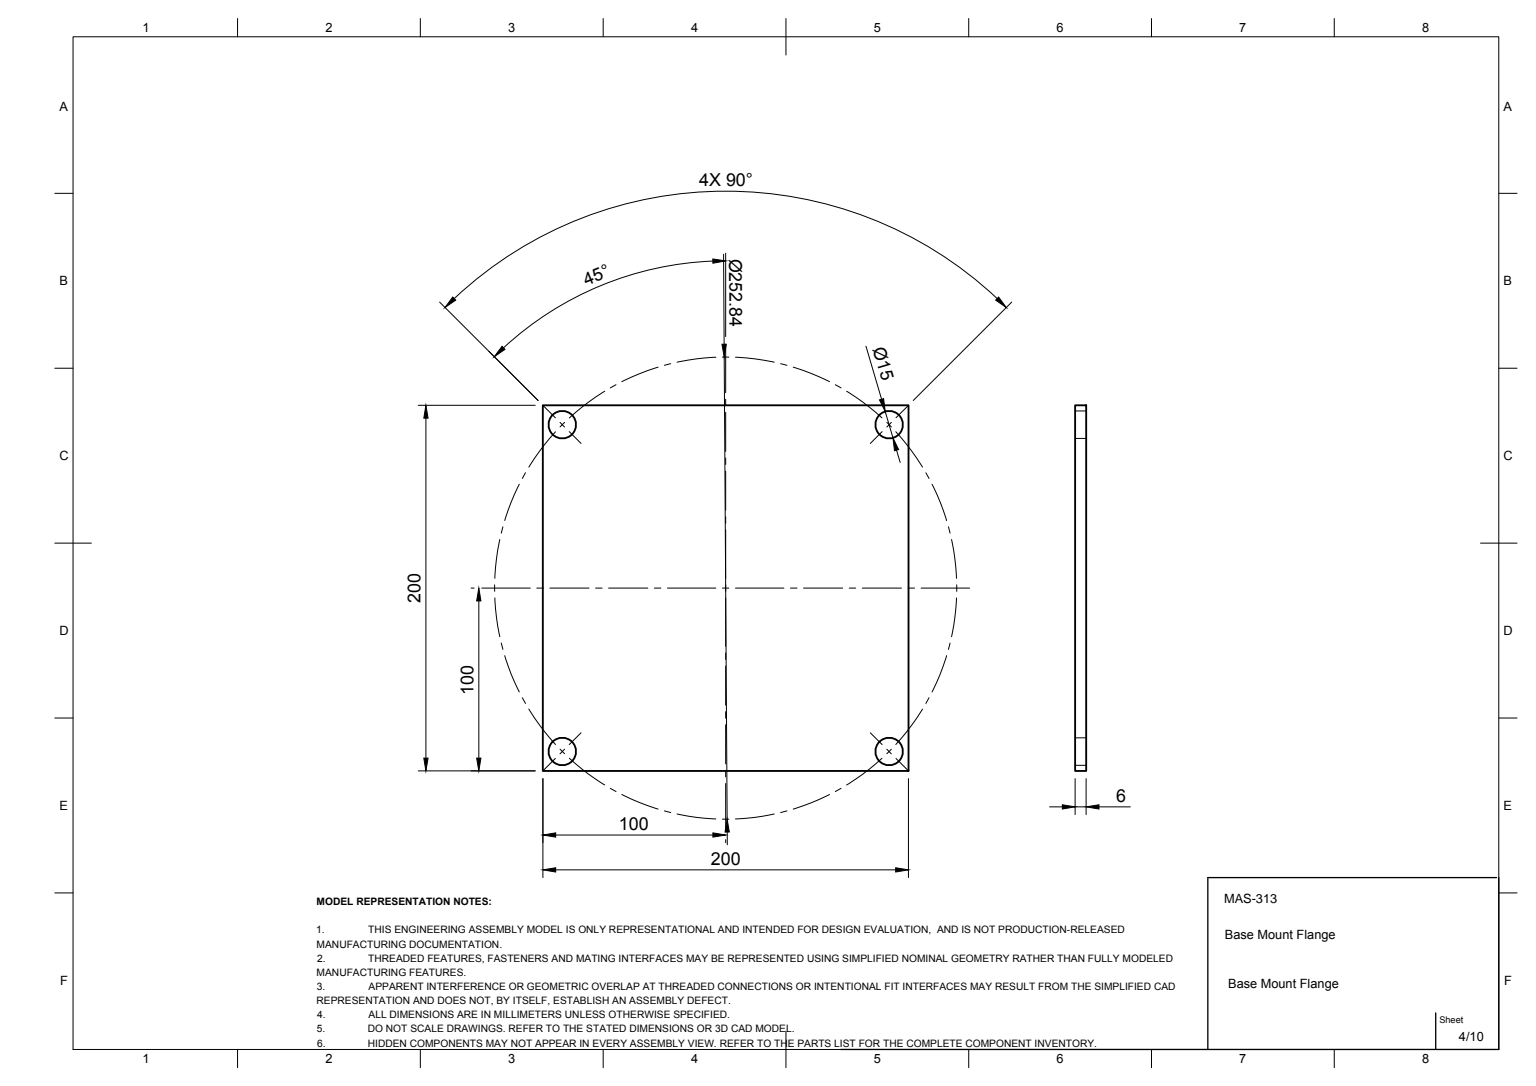
ISO-10303-21;
HEADER;
FILE_DESCRIPTION (('STEP AP214'),
    '1' );
FILE_NAME ('Base Mount Flange.step',
    '2026-10-06T09:36:00',
    ( '' ),
    ( '' ),
    'SwSTEP 2.0',
    'SolidWorks 2025',
    '' );
FILE_SCHEMA (( 'AUTOMOTIVE_DESIGN' ));
ENDSEC;

DATA;
#29=DIRECTION ( 'NONE',  ( 0.000000000000000000, 0.000000000000000000, 1.000000000000000000 ) ) ;
#31=CARTESIAN_POINT ( 'NONE',  ( 9.184850993605149917E-16, 0.000000000000000000, -133.9213562373095101 ) ) ;
#52=( NAMED_UNIT ( * ) PLANE_ANGLE_UNIT ( ) SI_UNIT ( $, .RADIAN. ) );
#69=VERTEX_POINT ( 'NONE', #7089 ) ;
#81=LINE ( 'NONE', #4059, #683 ) ;
#89=AXIS2_PLACEMENT_3D ( 'NONE', #10782, #5094, #8125 ) ;
#118=PRODUCT ( 'Base Mount Flange', 'Base Mount Flange', '', ( #4909 ) ) ;
#163=ORIENTED_EDGE ( 'NONE', *, *, #8870, .T. ) ;
#166=AXIS2_PLACEMENT_3D ( 'NONE', #11994, #9209, #3384 ) ;
#206=VERTEX_POINT ( 'NONE', #8210 ) ;
#238=EDGE_CURVE ( 'NONE', #2268, #7247, #10053, .T. ) ;
#269=DIRECTION ( 'NONE',  ( 0.000000000000000000, 0.000000000000000000, -1.000000000000000000 ) ) ;
#306=EDGE_LOOP ( 'NONE', ( #4987, #12037, #7872, #11168 ) ) ;
#325=ORIENTED_EDGE ( 'NONE', *, *, #5571, .T. ) ;
#336=LINE ( 'NONE', #1445, #8050 ) ;
#340=EDGE_CURVE ( 'NONE', #2669, #5042, #5605, .T. ) ;
#346=EDGE_LOOP ( 'NONE', ( #11443, #5040 ) ) ;
#365=ORIENTED_EDGE ( 'NONE', *, *, #10686, .T. ) ;
#368=VERTEX_POINT ( 'NONE', #31 ) ;
#387=ORIENTED_EDGE ( 'NONE', *, *, #9652, .F. ) ;
#405=CARTESIAN_POINT ( 'NONE',  ( 126.4213562373094959, -6.000000000000000000, -6.938893903907228378E-15 ) ) ;
#427=VECTOR ( 'NONE', #2802, 999.9999999999998863 ) ;
#471=ORIENTED_EDGE ( 'NONE', *, *, #4119, .T. ) ;
#534=DIRECTION ( 'NONE',  ( 0.000000000000000000, 1.000000000000000000, 0.000000000000000000 ) ) ;
#545=ORIENTED_EDGE ( 'NONE', *, *, #11311, .F. ) ;
#595=PLANE ( 'NONE',  #12120 ) ;
#617=DIRECTION ( 'NONE',  ( 0.000000000000000000, 1.000000000000000000, 0.000000000000000000 ) ) ;
#644=DIRECTION ( 'NONE',  ( 0.000000000000000000, 1.000000000000000000, 0.000000000000000000 ) ) ;
#667=CARTESIAN_POINT ( 'NONE',  ( -126.4213562373094959, -6.000000000000000000, -7.499999999999990230 ) ) ;
#683=VECTOR ( 'NONE', #11412, 1000.000000000000000 ) ;
#699=FACE_OUTER_BOUND ( 'NONE', #2730, .T. ) ;
#703=DIRECTION ( 'NONE',  ( -0.7071067811865479058, 0.000000000000000000, -0.7071067811865472397 ) ) ;
#715=CARTESIAN_POINT ( 'NONE',  ( 4.808665244885994618E-14, -6.000000000000000000, 141.4213562373094817 ) ) ;
#729=VECTOR ( 'NONE', #2030, 1000.000000000000000 ) ;
#742=CARTESIAN_POINT ( 'NONE',  ( 126.4213562373094959, -6.000000000000000000, -6.938893903907228378E-15 ) ) ;
#760=AXIS2_PLACEMENT_3D ( 'NONE', #9887, #5181, #11805 ) ;
#769=PLANE ( 'NONE',  #3066 ) ;
#771=PLANE ( 'NONE',  #1682 ) ;
#809=EDGE_LOOP ( 'NONE', ( #4329, #2289, #4115, #6023 ) ) ;
#811=CARTESIAN_POINT ( 'NONE',  ( 1.387778780781445676E-14, -6.000000000000000000, 126.4213562373094959 ) ) ;
#815=SURFACE_STYLE_FILL_AREA ( #9277 ) ;
#883=DIRECTION ( 'NONE',  ( 0.000000000000000000, 0.000000000000000000, -1.000000000000000000 ) ) ;
#885=CIRCLE ( 'NONE', #12132, 7.500000000000007105 ) ;
#951=ORIENTED_EDGE ( 'NONE', *, *, #3247, .T. ) ;
#967=VECTOR ( 'NONE', #6992, 999.9999999999998863 ) ;
#1130=VECTOR ( 'NONE', #12111, 1000.000000000000000 ) ;
#1133=EDGE_LOOP ( 'NONE', ( #5075, #8034, #10647, #2735 ) ) ;
#1141=ORIENTED_EDGE ( 'NONE', *, *, #8393, .T. ) ;
#1168=ADVANCED_FACE ( 'NONE', ( #10376 ), #7419, .F. ) ;
#1189=CIRCLE ( 'NONE', #4922, 7.500000000000007105 ) ;
#1219=VERTEX_POINT ( 'NONE', #9205 ) ;
#1274=AXIS2_PLACEMENT_3D ( 'NONE', #10202, #9278, #11130 ) ;
#1284=CIRCLE ( 'NONE', #89, 7.500000000000007105 ) ;
#1296=CYLINDRICAL_SURFACE ( 'NONE', #1870, 7.500000000000007105 ) ;
#1328=CARTESIAN_POINT ( 'NONE',  ( 4.808665244885994618E-14, 0.000000000000000000, 141.4213562373094817 ) ) ;
#1372=CIRCLE ( 'NONE', #166, 7.500000000000012434 ) ;
#1377=ADVANCED_FACE ( 'NONE', ( #9751 ), #1296, .F. ) ;
#1410=DIRECTION ( 'NONE',  ( 0.000000000000000000, 0.000000000000000000, 1.000000000000000000 ) ) ;
#1414=VERTEX_POINT ( 'NONE', #5983 ) ;
#1415=DIRECTION ( 'NONE',  ( 0.000000000000000000, 1.000000000000000000, 0.000000000000000000 ) ) ;
#1436=ORIENTED_EDGE ( 'NONE', *, *, #10649, .T. ) ;
#1445=CARTESIAN_POINT ( 'NONE',  ( 141.4213562373095101, -6.000000000000000000, -1.508194112741312283E-14 ) ) ;
#1629=FACE_OUTER_BOUND ( 'NONE', #9194, .T. ) ;
#1682=AXIS2_PLACEMENT_3D ( 'NONE', #5167, #3665, #703 ) ;
#1685=ADVANCED_FACE ( 'NONE', ( #9060 ), #595, .T. ) ;
#1690=VERTEX_POINT ( 'NONE', #10112 ) ;
#1794=EDGE_CURVE ( 'NONE', #6737, #10573, #4624, .T. ) ;
#1796=DIRECTION ( 'NONE',  ( 0.000000000000000000, 0.000000000000000000, 1.000000000000000000 ) ) ;
#1804=FACE_BOUND ( 'NONE', #4441, .T. ) ;
#1819=DIRECTION ( 'NONE',  ( 0.000000000000000000, 0.000000000000000000, 1.000000000000000000 ) ) ;
#1822=ORIENTED_EDGE ( 'NONE', *, *, #2939, .F. ) ;
#1828=DIRECTION ( 'NONE',  ( 0.000000000000000000, 0.000000000000000000, 1.000000000000000000 ) ) ;
#1835=VERTEX_POINT ( 'NONE', #2767 ) ;
#1851=CARTESIAN_POINT ( 'NONE',  ( -141.4213562373095101, 0.000000000000000000, 3.644282033693712520E-14 ) ) ;
#1870=AXIS2_PLACEMENT_3D ( 'NONE', #5794, #2163, #7715 ) ;
#1927=CIRCLE ( 'NONE', #5071, 7.500000000000012434 ) ;
#1946=ADVANCED_FACE ( 'NONE', ( #11248 ), #2636, .T. ) ;
#1961=CARTESIAN_POINT ( 'NONE',  ( 0.000000000000000000, -6.000000000000000000, -126.4213562373094959 ) ) ;
#2030=DIRECTION ( 'NONE',  ( 0.000000000000000000, 1.000000000000000000, 0.000000000000000000 ) ) ;
#2032=SHAPE_REPRESENTATION ( 'Base Mount Flange', ( #11957 ), #5231 ) ;
#2073=VERTEX_POINT ( 'NONE', #11418 ) ;
#2095=ORIENTED_EDGE ( 'NONE', *, *, #5571, .F. ) ;
#2107=CARTESIAN_POINT ( 'NONE',  ( 9.184850993605149917E-16, -6.000000000000000000, -133.9213562373095101 ) ) ;
#2136=CARTESIAN_POINT ( 'NONE',  ( 141.4213562373095101, 0.000000000000000000, -1.508194112741312283E-14 ) ) ;
#2163=DIRECTION ( 'NONE',  ( 0.000000000000000000, 1.000000000000000000, 0.000000000000000000 ) ) ;
#2173=VECTOR ( 'NONE', #8279, 1000.000000000000000 ) ;
#2217=DIRECTION ( 'NONE',  ( 0.000000000000000000, 1.000000000000000000, 0.000000000000000000 ) ) ;
#2252=ORIENTED_EDGE ( 'NONE', *, *, #3563, .F. ) ;
#2268=VERTEX_POINT ( 'NONE', #7013 ) ;
#2289=ORIENTED_EDGE ( 'NONE', *, *, #3136, .T. ) ;
#2296=LINE ( 'NONE', #4155, #967 ) ;
#2311=LINE ( 'NONE', #6080, #8141 ) ;
#2328=ORIENTED_EDGE ( 'NONE', *, *, #238, .T. ) ;
#2431=DIRECTION ( 'NONE',  ( -0.7071067811865479058, 0.000000000000000000, -0.7071067811865472397 ) ) ;
#2462=DIRECTION ( 'NONE',  ( 0.000000000000000000, 1.000000000000000000, 0.000000000000000000 ) ) ;
#2505=CARTESIAN_POINT ( 'NONE',  ( -126.4213562373094959, -6.000000000000000000, 2.255140518769849223E-14 ) ) ;
#2566=CYLINDRICAL_SURFACE ( 'NONE', #4120, 7.500000000000012434 ) ;
#2587=LINE ( 'NONE', #12124, #11929 ) ;
#2599=LINE ( 'NONE', #5733, #729 ) ;
#2629=CARTESIAN_POINT ( 'NONE',  ( 126.4213562373094959, -6.000000000000000000, 7.500000000000006217 ) ) ;
#2636=PLANE ( 'NONE',  #6970 ) ;
#2663=ORIENTED_EDGE ( 'NONE', *, *, #9249, .F. ) ;
#2669=VERTEX_POINT ( 'NONE', #9123 ) ;
#2676=DIRECTION ( 'NONE',  ( -0.7071067811865473507, 0.000000000000000000, 0.7071067811865477948 ) ) ;
#2711=CARTESIAN_POINT ( 'NONE',  ( 126.4213562373094959, -6.000000000000000000, 7.500000000000006217 ) ) ;
#2714=VECTOR ( 'NONE', #1415, 1000.000000000000000 ) ;
#2723=CARTESIAN_POINT ( 'NONE',  ( 0.000000000000000000, 0.000000000000000000, -126.4213562373094959 ) ) ;
#2730=EDGE_LOOP ( 'NONE', ( #5594, #2095, #163, #11247 ) ) ;
#2735=ORIENTED_EDGE ( 'NONE', *, *, #11986, .F. ) ;
#2754=DIRECTION ( 'NONE',  ( 0.000000000000000000, 1.000000000000000000, 0.000000000000000000 ) ) ;
#2762=EDGE_LOOP ( 'NONE', ( #10234, #2252 ) ) ;
#2767=CARTESIAN_POINT ( 'NONE',  ( -126.4213562373094959, -6.000000000000000000, -7.499999999999990230 ) ) ;
#2802=DIRECTION ( 'NONE',  ( -0.7071067811865473507, -0.000000000000000000, 0.7071067811865477948 ) ) ;
#2807=VECTOR ( 'NONE', #2462, 1000.000000000000000 ) ;
#2846=DIRECTION ( 'NONE',  ( 0.000000000000000000, 0.000000000000000000, 1.000000000000000000 ) ) ;
#2939=EDGE_CURVE ( 'NONE', #206, #8172, #3231, .T. ) ;
#3065=FACE_BOUND ( 'NONE', #5038, .T. ) ;
#3066=AXIS2_PLACEMENT_3D ( 'NONE', #11833, #5521, #2676 ) ;
#3084=CARTESIAN_POINT ( 'NONE',  ( -6.360897667028196044E-14, 0.000000000000000000, -141.4213562373094817 ) ) ;
#3136=EDGE_CURVE ( 'NONE', #69, #7247, #2587, .T. ) ;
#3155=EDGE_CURVE ( 'NONE', #7478, #12001, #7190, .T. ) ;
#3231=CIRCLE ( 'NONE', #6397, 7.500000000000007105 ) ;
#3247=EDGE_CURVE ( 'NONE', #1219, #5163, #7881, .T. ) ;
#3250=VECTOR ( 'NONE', #10946, 1000.000000000000000 ) ;
#3347=ORIENTED_EDGE ( 'NONE', *, *, #6546, .T. ) ;
#3384=DIRECTION ( 'NONE',  ( 0.000000000000000000, 0.000000000000000000, 1.000000000000000000 ) ) ;
#3407=CARTESIAN_POINT ( 'NONE',  ( 1.387778780781445676E-14, -6.000000000000000000, 133.9213562373095101 ) ) ;
#3415=ADVANCED_FACE ( 'NONE', ( #4015 ), #11558, .F. ) ;
#3434=VERTEX_POINT ( 'NONE', #3084 ) ;
#3475=DIRECTION ( 'NONE',  ( 0.000000000000000000, 1.000000000000000000, 0.000000000000000000 ) ) ;
#3495=ORIENTED_EDGE ( 'NONE', *, *, #4816, .F. ) ;
#3527=FACE_OUTER_BOUND ( 'NONE', #5714, .T. ) ;
#3534=DIRECTION ( 'NONE',  ( 0.000000000000000000, 0.000000000000000000, 1.000000000000000000 ) ) ;
#3550=ADVANCED_FACE ( 'NONE', ( #10986 ), #9752, .F. ) ;
#3563=EDGE_CURVE ( 'NONE', #1690, #5876, #6103, .T. ) ;
#3572=FACE_BOUND ( 'NONE', #2762, .T. ) ;
#3638=PRESENTATION_STYLE_ASSIGNMENT (( #8363 ) ) ;
#3665=DIRECTION ( 'NONE',  ( 0.7071067811865472397, 0.000000000000000000, -0.7071067811865479058 ) ) ;
#3670=PRODUCT_DEFINITION_FORMATION_WITH_SPECIFIED_SOURCE ( 'ANY', '', #118, .NOT_KNOWN. ) ;
#3691=EDGE_LOOP ( 'NONE', ( #9564, #6137, #10492, #8006 ) ) ;
#3709=CARTESIAN_POINT ( 'NONE',  ( -126.4213562373094959, -6.000000000000000000, 7.500000000000035527 ) ) ;
#3763=ORIENTED_EDGE ( 'NONE', *, *, #3155, .T. ) ;
#3769=( NAMED_UNIT ( * ) SI_UNIT ( $, .STERADIAN. ) SOLID_ANGLE_UNIT ( ) );
#3801=ORIENTED_EDGE ( 'NONE', *, *, #4816, .T. ) ;
#3803=EDGE_CURVE ( 'NONE', #5876, #1690, #5511, .T. ) ;
#3822=EDGE_CURVE ( 'NONE', #12001, #7478, #1372, .T. ) ;
#3860=MANIFOLD_SOLID_BREP ( 'Boss-Extrude1', #8083 ) ;
#3934=CARTESIAN_POINT ( 'NONE',  ( 0.000000000000000000, -6.000000000000000000, 0.000000000000000000 ) ) ;
#3960=ORIENTED_EDGE ( 'NONE', *, *, #10605, .F. ) ;
#3961=ORIENTED_EDGE ( 'NONE', *, *, #1794, .F. ) ;
#4015=FACE_OUTER_BOUND ( 'NONE', #7902, .T. ) ;
#4034=CIRCLE ( 'NONE', #1274, 7.500000000000012434 ) ;
#4059=CARTESIAN_POINT ( 'NONE',  ( 9.184850993605153861E-16, -6.000000000000000000, -133.9213562373095101 ) ) ;
#4071=ORIENTED_EDGE ( 'NONE', *, *, #4965, .T. ) ;
#4115=ORIENTED_EDGE ( 'NONE', *, *, #5783, .T. ) ;
#4119=EDGE_CURVE ( 'NONE', #10573, #6737, #1189, .T. ) ;
#4120=AXIS2_PLACEMENT_3D ( 'NONE', #2505, #7209, #7399 ) ;
#4155=CARTESIAN_POINT ( 'NONE',  ( -141.4213562373095101, -6.000000000000000000, 3.644282033693712520E-14 ) ) ;
#4161=DIRECTION ( 'NONE',  ( 0.000000000000000000, 1.000000000000000000, 0.000000000000000000 ) ) ;
#4163=ORIENTED_EDGE ( 'NONE', *, *, #11692, .T. ) ;
#4329=ORIENTED_EDGE ( 'NONE', *, *, #7278, .T. ) ;
#4361=ADVANCED_FACE ( 'NONE', ( #7270 ), #2566, .F. ) ;
#4394=FACE_BOUND ( 'NONE', #11723, .T. ) ;
#4441=EDGE_LOOP ( 'NONE', ( #6502, #4537 ) ) ;
#4464=CARTESIAN_POINT ( 'NONE',  ( -126.4213562373094959, 0.000000000000000000, -7.499999999999990230 ) ) ;
#4475=CIRCLE ( 'NONE', #11381, 7.500000000000012434 ) ;
#4493=CIRCLE ( 'NONE', #7846, 7.500000000000012434 ) ;
#4520=DIRECTION ( 'NONE',  ( 0.000000000000000000, 1.000000000000000000, 0.000000000000000000 ) ) ;
#4537=ORIENTED_EDGE ( 'NONE', *, *, #6350, .F. ) ;
#4587=SURFACE_SIDE_STYLE ('',( #815 ) ) ;
#4599=ADVANCED_FACE ( 'NONE', ( #4746 ), #4912, .F. ) ;
#4624=CIRCLE ( 'NONE', #11521, 7.500000000000007105 ) ;
#4746=FACE_OUTER_BOUND ( 'NONE', #9447, .T. ) ;
#4759=CARTESIAN_POINT ( 'NONE',  ( 0.000000000000000000, -6.000000000000000000, -126.4213562373094959 ) ) ;
#4777=DIRECTION ( 'NONE',  ( 0.000000000000000000, 0.000000000000000000, 1.000000000000000000 ) ) ;
#4816=EDGE_CURVE ( 'NONE', #5163, #7478, #5475, .T. ) ;
#4823=AXIS2_PLACEMENT_3D ( 'NONE', #9717, #5069, #5011 ) ;
#4854=PLANE ( 'NONE',  #6567 ) ;
#4906=DIRECTION ( 'NONE',  ( 0.7071067811865479058, -0.000000000000000000, 0.7071067811865472397 ) ) ;
#4909=PRODUCT_CONTEXT ( 'NONE', #9295, 'mechanical' ) ;
#4912=CYLINDRICAL_SURFACE ( 'NONE', #9238, 7.500000000000007105 ) ;
#4914=FACE_OUTER_BOUND ( 'NONE', #1133, .T. ) ;
#4922=AXIS2_PLACEMENT_3D ( 'NONE', #9968, #7060, #10831 ) ;
#4951=ORIENTED_EDGE ( 'NONE', *, *, #11986, .T. ) ;
#4965=EDGE_CURVE ( 'NONE', #1219, #12001, #6919, .T. ) ;
#4974=UNCERTAINTY_MEASURE_WITH_UNIT (LENGTH_MEASURE( 1.000000000000000082E-05 ), #8426, 'distance_accuracy_value', 'NONE');
#4977=AXIS2_PLACEMENT_3D ( 'NONE', #11946, #7318, #1819 ) ;
#4982=ORIENTED_EDGE ( 'NONE', *, *, #6350, .T. ) ;
#4987=ORIENTED_EDGE ( 'NONE', *, *, #7278, .F. ) ;
#5011=DIRECTION ( 'NONE',  ( 0.000000000000000000, 0.000000000000000000, 1.000000000000000000 ) ) ;
#5018=CARTESIAN_POINT ( 'NONE',  ( -126.4213562373094959, 0.000000000000000000, 2.255140518769849223E-14 ) ) ;
#5038=EDGE_LOOP ( 'NONE', ( #1141, #5808 ) ) ;
#5040=ORIENTED_EDGE ( 'NONE', *, *, #2939, .T. ) ;
#5042=VERTEX_POINT ( 'NONE', #8037 ) ;
#5057=DIRECTION ( 'NONE',  ( 0.000000000000000000, 1.000000000000000000, 0.000000000000000000 ) ) ;
#5069=DIRECTION ( 'NONE',  ( 0.000000000000000000, 1.000000000000000000, 0.000000000000000000 ) ) ;
#5071=AXIS2_PLACEMENT_3D ( 'NONE', #11029, #10100, #1828 ) ;
#5075=ORIENTED_EDGE ( 'NONE', *, *, #340, .F. ) ;
#5094=DIRECTION ( 'NONE',  ( 0.000000000000000000, 1.000000000000000000, 0.000000000000000000 ) ) ;
#5101=AXIS2_PLACEMENT_3D ( 'NONE', #11005, #6309, #883 ) ;
#5108=AXIS2_PLACEMENT_3D ( 'NONE', #4759, #2217, #6912 ) ;
#5161=ORIENTED_EDGE ( 'NONE', *, *, #4119, .F. ) ;
#5163=VERTEX_POINT ( 'NONE', #2711 ) ;
#5167=CARTESIAN_POINT ( 'NONE',  ( 141.4213562373095101, -6.000000000000000000, -1.508194112741312283E-14 ) ) ;
#5177=DIRECTION ( 'NONE',  ( 0.000000000000000000, 1.000000000000000000, 0.000000000000000000 ) ) ;
#5181=DIRECTION ( 'NONE',  ( 0.000000000000000000, 1.000000000000000000, 0.000000000000000000 ) ) ;
#5231=( GEOMETRIC_REPRESENTATION_CONTEXT ( 3 ) GLOBAL_UNCERTAINTY_ASSIGNED_CONTEXT ( ( #6835 ) ) GLOBAL_UNIT_ASSIGNED_CONTEXT ( ( #7077, #7202, #5973 ) ) REPRESENTATION_CONTEXT ( 'NONE', 'WORKASPACE' ) );
#5448=ORIENTED_EDGE ( 'NONE', *, *, #1794, .T. ) ;
#5475=LINE ( 'NONE', #2629, #7131 ) ;
#5494=EDGE_LOOP ( 'NONE', ( #11595, #3960, #4951, #2328 ) ) ;
#5511=CIRCLE ( 'NONE', #12235, 7.500000000000007105 ) ;
#5516=ORIENTED_EDGE ( 'NONE', *, *, #10153, .T. ) ;
#5521=DIRECTION ( 'NONE',  ( -0.7071067811865477948, 0.000000000000000000, -0.7071067811865473507 ) ) ;
#5536=LINE ( 'NONE', #11237, #11392 ) ;
#5540=DIRECTION ( 'NONE',  ( -0.7071067811865472397, 0.000000000000000000, 0.7071067811865479058 ) ) ;
#5551=EDGE_LOOP ( 'NONE', ( #11276, #10366, #9344, #2663 ) ) ;
#5571=EDGE_CURVE ( 'NONE', #5951, #3434, #8098, .T. ) ;
#5594=ORIENTED_EDGE ( 'NONE', *, *, #5948, .F. ) ;
#5605=LINE ( 'NONE', #7403, #6512 ) ;
#5609=DIRECTION ( 'NONE',  ( 0.7071067811865477948, -0.000000000000000000, 0.7071067811865473507 ) ) ;
#5695=ADVANCED_FACE ( 'NONE', ( #3065, #6768, #9678, #10542, #4914 ), #4854, .T. ) ;
#5714=EDGE_LOOP ( 'NONE', ( #8458, #4071, #9918, #3495 ) ) ;
#5733=CARTESIAN_POINT ( 'NONE',  ( 1.479627290717497352E-14, -6.000000000000000000, 118.9213562373094817 ) ) ;
#5737=EDGE_LOOP ( 'NONE', ( #471, #5448 ) ) ;
#5783=EDGE_CURVE ( 'NONE', #7247, #3434, #2311, .T. ) ;
#5794=CARTESIAN_POINT ( 'NONE',  ( 1.387778780781445676E-14, -6.000000000000000000, 126.4213562373094959 ) ) ;
#5808=ORIENTED_EDGE ( 'NONE', *, *, #6542, .T. ) ;
#5876=VERTEX_POINT ( 'NONE', #10031 ) ;
#5896=AXIS2_PLACEMENT_3D ( 'NONE', #742, #4520, #2846 ) ;
#5932=CYLINDRICAL_SURFACE ( 'NONE', #8048, 7.500000000000012434 ) ;
#5933=ADVANCED_FACE ( 'NONE', ( #3527 ), #12008, .F. ) ;
#5939=EDGE_LOOP ( 'NONE', ( #10719, #387 ) ) ;
#5948=EDGE_CURVE ( 'NONE', #3434, #8433, #8179, .T. ) ;
#5951=VERTEX_POINT ( 'NONE', #11017 ) ;
#5973=( NAMED_UNIT ( * ) SI_UNIT ( $, .STERADIAN. ) SOLID_ANGLE_UNIT ( ) );
#5983=CARTESIAN_POINT ( 'NONE',  ( 0.000000000000000000, 0.000000000000000000, -118.9213562373094817 ) ) ;
#6023=ORIENTED_EDGE ( 'NONE', *, *, #5948, .T. ) ;
#6080=CARTESIAN_POINT ( 'NONE',  ( 141.4213562373095101, 0.000000000000000000, -1.508194112741312283E-14 ) ) ;
#6103=CIRCLE ( 'NONE', #6884, 7.500000000000007105 ) ;
#6113=CARTESIAN_POINT ( 'NONE',  ( 1.387778780781445676E-14, 0.000000000000000000, 126.4213562373094959 ) ) ;
#6137=ORIENTED_EDGE ( 'NONE', *, *, #8393, .F. ) ;
#6307=CARTESIAN_POINT ( 'NONE',  ( 0.000000000000000000, -6.000000000000000000, -118.9213562373094817 ) ) ;
#6308=ORIENTED_EDGE ( 'NONE', *, *, #5783, .F. ) ;
#6309=DIRECTION ( 'NONE',  ( 0.000000000000000000, -1.000000000000000000, 0.000000000000000000 ) ) ;
#6333=CARTESIAN_POINT ( 'NONE',  ( 126.4213562373094959, 0.000000000000000000, -7.500000000000019540 ) ) ;
#6338=DIRECTION ( 'NONE',  ( 0.000000000000000000, 0.000000000000000000, 1.000000000000000000 ) ) ;
#6350=EDGE_CURVE ( 'NONE', #368, #1414, #11333, .T. ) ;
#6397=AXIS2_PLACEMENT_3D ( 'NONE', #7373, #9291, #4777 ) ;
#6502=ORIENTED_EDGE ( 'NONE', *, *, #6546, .F. ) ;
#6512=VECTOR ( 'NONE', #9382, 999.9999999999998863 ) ;
#6542=EDGE_CURVE ( 'NONE', #1835, #11782, #4034, .T. ) ;
#6546=EDGE_CURVE ( 'NONE', #1414, #368, #885, .T. ) ;
#6567=AXIS2_PLACEMENT_3D ( 'NONE', #3934, #7763, #269 ) ;
#6592=CARTESIAN_POINT ( 'NONE',  ( 0.000000000000000000, -6.000000000000000000, -126.4213562373094959 ) ) ;
#6605=AXIS2_PLACEMENT_3D ( 'NONE', #12189, #10131, #1796 ) ;
#6635=ORIENTED_EDGE ( 'NONE', *, *, #11042, .T. ) ;
#6737=VERTEX_POINT ( 'NONE', #2107 ) ;
#6768=FACE_BOUND ( 'NONE', #346, .T. ) ;
#6835=UNCERTAINTY_MEASURE_WITH_UNIT (LENGTH_MEASURE( 1.000000000000000082E-05 ), #7077, 'distance_accuracy_value', 'NONE');
#6884=AXIS2_PLACEMENT_3D ( 'NONE', #6113, #534, #1410 ) ;
#6894=( GEOMETRIC_REPRESENTATION_CONTEXT ( 3 ) GLOBAL_UNCERTAINTY_ASSIGNED_CONTEXT ( ( #4974 ) ) GLOBAL_UNIT_ASSIGNED_CONTEXT ( ( #8426, #52, #3769 ) ) REPRESENTATION_CONTEXT ( 'NONE', 'WORKASPACE' ) );
#6912=DIRECTION ( 'NONE',  ( 0.000000000000000000, 0.000000000000000000, 1.000000000000000000 ) ) ;
#6919=LINE ( 'NONE', #11685, #10691 ) ;
#6945=DIRECTION ( 'NONE',  ( -0.7071067811865479058, 0.000000000000000000, -0.7071067811865472397 ) ) ;
#6957=CARTESIAN_POINT ( 'NONE',  ( 4.808665244885994618E-14, -6.000000000000000000, 141.4213562373094817 ) ) ;
#6970=AXIS2_PLACEMENT_3D ( 'NONE', #9256, #5609, #9385 ) ;
#6992=DIRECTION ( 'NONE',  ( -0.7071067811865473507, -0.000000000000000000, 0.7071067811865477948 ) ) ;
#7013=CARTESIAN_POINT ( 'NONE',  ( 141.4213562373095101, -6.000000000000000000, -1.508194112741312283E-14 ) ) ;
#7060=DIRECTION ( 'NONE',  ( 0.000000000000000000, 1.000000000000000000, 0.000000000000000000 ) ) ;
#7077=( LENGTH_UNIT ( ) NAMED_UNIT ( * ) SI_UNIT ( .MILLI., .METRE. ) );
#7089=CARTESIAN_POINT ( 'NONE',  ( 4.808665244885994618E-14, 0.000000000000000000, 141.4213562373094817 ) ) ;
#7099=LINE ( 'NONE', #9884, #2714 ) ;
#7131=VECTOR ( 'NONE', #7150, 1000.000000000000000 ) ;
#7144=DIRECTION ( 'NONE',  ( 0.7071067811865473507, 0.000000000000000000, -0.7071067811865477948 ) ) ;
#7150=DIRECTION ( 'NONE',  ( 0.000000000000000000, 1.000000000000000000, 0.000000000000000000 ) ) ;
#7158=APPLICATION_CONTEXT ( 'automotive_design' ) ;
#7161=FACE_OUTER_BOUND ( 'NONE', #5551, .T. ) ;
#7186=EDGE_LOOP ( 'NONE', ( #1822, #5516, #12129, #9492 ) ) ;
#7190=CIRCLE ( 'NONE', #6605, 7.500000000000012434 ) ;
#7202=( NAMED_UNIT ( * ) PLANE_ANGLE_UNIT ( ) SI_UNIT ( $, .RADIAN. ) );
#7209=DIRECTION ( 'NONE',  ( 0.000000000000000000, 1.000000000000000000, 0.000000000000000000 ) ) ;
#7236=DIRECTION ( 'NONE',  ( 0.000000000000000000, 0.000000000000000000, 1.000000000000000000 ) ) ;
#7247=VERTEX_POINT ( 'NONE', #2136 ) ;
#7252=CARTESIAN_POINT ( 'NONE',  ( -141.4213562373095101, 0.000000000000000000, 3.644282033693712520E-14 ) ) ;
#7270=FACE_OUTER_BOUND ( 'NONE', #3691, .T. ) ;
#7278=EDGE_CURVE ( 'NONE', #8433, #69, #7755, .T. ) ;
#7318=DIRECTION ( 'NONE',  ( 0.000000000000000000, 1.000000000000000000, 0.000000000000000000 ) ) ;
#7373=CARTESIAN_POINT ( 'NONE',  ( 1.387778780781445676E-14, -6.000000000000000000, 126.4213562373094959 ) ) ;
#7399=DIRECTION ( 'NONE',  ( 0.000000000000000000, 0.000000000000000000, 1.000000000000000000 ) ) ;
#7403=CARTESIAN_POINT ( 'NONE',  ( 4.808665244885994618E-14, -6.000000000000000000, 141.4213562373094817 ) ) ;
#7419=CYLINDRICAL_SURFACE ( 'NONE', #7549, 7.500000000000007105 ) ;
#7478=VERTEX_POINT ( 'NONE', #10459 ) ;
#7493=STYLED_ITEM ( 'NONE', ( #3638 ), #3860 ) ;
#7549=AXIS2_PLACEMENT_3D ( 'NONE', #811, #9455, #9272 ) ;
#7643=ADVANCED_FACE ( 'NONE', ( #1629 ), #771, .T. ) ;
#7649=VECTOR ( 'NONE', #2754, 1000.000000000000000 ) ;
#7715=DIRECTION ( 'NONE',  ( 0.000000000000000000, 0.000000000000000000, 1.000000000000000000 ) ) ;
#7722=EDGE_LOOP ( 'NONE', ( #12009, #10107, #3801, #3763 ) ) ;
#7743=ORIENTED_EDGE ( 'NONE', *, *, #11042, .F. ) ;
#7744=ADVANCED_FACE ( 'NONE', ( #699 ), #769, .T. ) ;
#7755=LINE ( 'NONE', #1328, #7799 ) ;
#7763=DIRECTION ( 'NONE',  ( 0.000000000000000000, -1.000000000000000000, 0.000000000000000000 ) ) ;
#7799=VECTOR ( 'NONE', #4906, 999.9999999999998863 ) ;
#7846=AXIS2_PLACEMENT_3D ( 'NONE', #11092, #3475, #3534 ) ;
#7872=ORIENTED_EDGE ( 'NONE', *, *, #340, .T. ) ;
#7876=DIRECTION ( 'NONE',  ( 0.000000000000000000, 0.000000000000000000, 1.000000000000000000 ) ) ;
#7881=CIRCLE ( 'NONE', #5896, 7.500000000000012434 ) ;
#7902=EDGE_LOOP ( 'NONE', ( #3961, #6635, #4982, #11844 ) ) ;
#7955=DIRECTION ( 'NONE',  ( 1.000000000000000000, 0.000000000000000000, 0.000000000000000000 ) ) ;
#8006=ORIENTED_EDGE ( 'NONE', *, *, #10735, .T. ) ;
#8009=VECTOR ( 'NONE', #7144, 999.9999999999998863 ) ;
#8034=ORIENTED_EDGE ( 'NONE', *, *, #8870, .F. ) ;
#8037=CARTESIAN_POINT ( 'NONE',  ( 4.808665244885994618E-14, -6.000000000000000000, 141.4213562373094817 ) ) ;
#8048=AXIS2_PLACEMENT_3D ( 'NONE', #8833, #5177, #10747 ) ;
#8050=VECTOR ( 'NONE', #2431, 999.9999999999998863 ) ;
#8083=CLOSED_SHELL ( 'NONE', ( #9154, #1168, #5933, #3415, #1685, #7744, #7643, #1946, #5695, #9029, #4599, #3550, #1377, #4361 ) ) ;
#8098=LINE ( 'NONE', #10933, #2807 ) ;
#8125=DIRECTION ( 'NONE',  ( 0.000000000000000000, 0.000000000000000000, 1.000000000000000000 ) ) ;
#8141=VECTOR ( 'NONE', #6945, 999.9999999999998863 ) ;
#8172=VERTEX_POINT ( 'NONE', #11071 ) ;
#8179=LINE ( 'NONE', #7252, #427 ) ;
#8210=CARTESIAN_POINT ( 'NONE',  ( 1.479627290717497352E-14, -6.000000000000000000, 118.9213562373094817 ) ) ;
#8239=FACE_BOUND ( 'NONE', #5939, .T. ) ;
#8248=VECTOR ( 'NONE', #644, 1000.000000000000000 ) ;
#8279=DIRECTION ( 'NONE',  ( 0.000000000000000000, 1.000000000000000000, 0.000000000000000000 ) ) ;
#8304=LINE ( 'NONE', #6307, #3250 ) ;
#8363=SURFACE_STYLE_USAGE ( .BOTH. , #4587 ) ;
#8393=EDGE_CURVE ( 'NONE', #11782, #1835, #11814, .T. ) ;
#8426=( LENGTH_UNIT ( ) NAMED_UNIT ( * ) SI_UNIT ( .MILLI., .METRE. ) );
#8433=VERTEX_POINT ( 'NONE', #1851 ) ;
#8458=ORIENTED_EDGE ( 'NONE', *, *, #3247, .F. ) ;
#8516=DIRECTION ( 'NONE',  ( 0.000000000000000000, 1.000000000000000000, 0.000000000000000000 ) ) ;
#8823=CARTESIAN_POINT ( 'NONE',  ( 4.808665244885994618E-14, -6.000000000000000000, 141.4213562373094817 ) ) ;
#8830=DIRECTION ( 'NONE',  ( 0.000000000000000000, 1.000000000000000000, 0.000000000000000000 ) ) ;
#8833=CARTESIAN_POINT ( 'NONE',  ( -126.4213562373094959, -6.000000000000000000, 2.255140518769849223E-14 ) ) ;
#8841=ADVANCED_BREP_SHAPE_REPRESENTATION ( '', ( #3860, #11957 ), #5231 ) ;
#8866=COLOUR_RGB ( '', 0.31764706, 0.68627451, 0.89019608) ;
#8870=EDGE_CURVE ( 'NONE', #5951, #2669, #2296, .T. ) ;
#9029=ADVANCED_FACE ( 'NONE', ( #8239, #3572, #4394, #1804, #12195 ), #11070, .F. ) ;
#9032=ORIENTED_EDGE ( 'NONE', *, *, #10153, .F. ) ;
#9048=CARTESIAN_POINT ( 'NONE',  ( 0.000000000000000000, 0.000000000000000000, 0.000000000000000000 ) ) ;
#9057=MECHANICAL_DESIGN_GEOMETRIC_PRESENTATION_REPRESENTATION('',(#7493),#6894);
#9060=FACE_OUTER_BOUND ( 'NONE', #306, .T. ) ;
#9121=CARTESIAN_POINT ( 'NONE',  ( 141.4213562373095101, -6.000000000000000000, -1.508194112741312283E-14 ) ) ;
#9123=CARTESIAN_POINT ( 'NONE',  ( -141.4213562373095101, -6.000000000000000000, 3.644282033693712520E-14 ) ) ;
#9154=ADVANCED_FACE ( 'NONE', ( #7161 ), #5932, .F. ) ;
#9194=EDGE_LOOP ( 'NONE', ( #6308, #12003, #10309, #325 ) ) ;
#9205=CARTESIAN_POINT ( 'NONE',  ( 126.4213562373094959, -6.000000000000000000, -7.500000000000019540 ) ) ;
#9209=DIRECTION ( 'NONE',  ( 0.000000000000000000, 1.000000000000000000, 0.000000000000000000 ) ) ;
#9238=AXIS2_PLACEMENT_3D ( 'NONE', #1961, #8516, #29 ) ;
#9249=EDGE_CURVE ( 'NONE', #11782, #2073, #7099, .T. ) ;
#9256=CARTESIAN_POINT ( 'NONE',  ( 4.808665244885994618E-14, -6.000000000000000000, 141.4213562373094817 ) ) ;
#9272=DIRECTION ( 'NONE',  ( 0.000000000000000000, 0.000000000000000000, 1.000000000000000000 ) ) ;
#9277=FILL_AREA_STYLE ('',( #10201 ) ) ;
#9278=DIRECTION ( 'NONE',  ( 0.000000000000000000, 1.000000000000000000, 0.000000000000000000 ) ) ;
#9291=DIRECTION ( 'NONE',  ( 0.000000000000000000, 1.000000000000000000, 0.000000000000000000 ) ) ;
#9295=APPLICATION_CONTEXT ( 'automotive_design' ) ;
#9344=ORIENTED_EDGE ( 'NONE', *, *, #9652, .T. ) ;
#9382=DIRECTION ( 'NONE',  ( 0.7071067811865479058, -0.000000000000000000, 0.7071067811865472397 ) ) ;
#9385=DIRECTION ( 'NONE',  ( 0.7071067811865473507, 0.000000000000000000, -0.7071067811865477948 ) ) ;
#9392=EDGE_CURVE ( 'NONE', #1835, #10209, #10060, .T. ) ;
#9447=EDGE_LOOP ( 'NONE', ( #7743, #5161, #4163, #3347 ) ) ;
#9455=DIRECTION ( 'NONE',  ( 0.000000000000000000, 1.000000000000000000, 0.000000000000000000 ) ) ;
#9489=SHAPE_DEFINITION_REPRESENTATION ( #10493, #2032 ) ;
#9492=ORIENTED_EDGE ( 'NONE', *, *, #10686, .F. ) ;
#9564=ORIENTED_EDGE ( 'NONE', *, *, #9392, .F. ) ;
#9652=EDGE_CURVE ( 'NONE', #10209, #2073, #4475, .T. ) ;
#9678=FACE_BOUND ( 'NONE', #11435, .T. ) ;
#9717=CARTESIAN_POINT ( 'NONE',  ( 0.000000000000000000, 0.000000000000000000, -126.4213562373094959 ) ) ;
#9751=FACE_OUTER_BOUND ( 'NONE', #10599, .T. ) ;
#9752=CYLINDRICAL_SURFACE ( 'NONE', #11027, 7.500000000000012434 ) ;
#9884=CARTESIAN_POINT ( 'NONE',  ( -126.4213562373094959, -6.000000000000000000, 7.500000000000035527 ) ) ;
#9887=CARTESIAN_POINT ( 'NONE',  ( -126.4213562373094959, -6.000000000000000000, 2.255140518769849223E-14 ) ) ;
#9918=ORIENTED_EDGE ( 'NONE', *, *, #3822, .T. ) ;
#9935=PRODUCT_DEFINITION ( 'UNKNOWN', '', #3670, #11477 ) ;
#9968=CARTESIAN_POINT ( 'NONE',  ( 0.000000000000000000, -6.000000000000000000, -126.4213562373094959 ) ) ;
#10031=CARTESIAN_POINT ( 'NONE',  ( 1.387778780781445676E-14, 0.000000000000000000, 133.9213562373095101 ) ) ;
#10053=LINE ( 'NONE', #9121, #2173 ) ;
#10060=LINE ( 'NONE', #667, #1130 ) ;
#10064=EDGE_CURVE ( 'NONE', #2669, #8433, #5536, .T. ) ;
#10072=DIRECTION ( 'NONE',  ( 0.000000000000000000, 0.000000000000000000, 1.000000000000000000 ) ) ;
#10100=DIRECTION ( 'NONE',  ( 0.000000000000000000, 1.000000000000000000, 0.000000000000000000 ) ) ;
#10107=ORIENTED_EDGE ( 'NONE', *, *, #10649, .F. ) ;
#10112=CARTESIAN_POINT ( 'NONE',  ( 1.479627290717497352E-14, 0.000000000000000000, 118.9213562373094817 ) ) ;
#10131=DIRECTION ( 'NONE',  ( 0.000000000000000000, 1.000000000000000000, 0.000000000000000000 ) ) ;
#10153=EDGE_CURVE ( 'NONE', #206, #1690, #2599, .T. ) ;
#10201=FILL_AREA_STYLE_COLOUR ( '', #8866 ) ;
#10202=CARTESIAN_POINT ( 'NONE',  ( -126.4213562373094959, -6.000000000000000000, 2.255140518769849223E-14 ) ) ;
#10209=VERTEX_POINT ( 'NONE', #4464 ) ;
#10234=ORIENTED_EDGE ( 'NONE', *, *, #3803, .F. ) ;
#10239=DIRECTION ( 'NONE',  ( 0.000000000000000000, 1.000000000000000000, 0.000000000000000000 ) ) ;
#10250=ORIENTED_EDGE ( 'NONE', *, *, #3155, .F. ) ;
#10309=ORIENTED_EDGE ( 'NONE', *, *, #10564, .T. ) ;
#10366=ORIENTED_EDGE ( 'NONE', *, *, #9392, .T. ) ;
#10376=FACE_OUTER_BOUND ( 'NONE', #7186, .T. ) ;
#10459=CARTESIAN_POINT ( 'NONE',  ( 126.4213562373094959, 0.000000000000000000, 7.500000000000006217 ) ) ;
#10492=ORIENTED_EDGE ( 'NONE', *, *, #9249, .T. ) ;
#10493=PRODUCT_DEFINITION_SHAPE ( 'NONE', 'NONE',  #9935 ) ;
#10542=FACE_BOUND ( 'NONE', #5737, .T. ) ;
#10564=EDGE_CURVE ( 'NONE', #2268, #5951, #336, .T. ) ;
#10573=VERTEX_POINT ( 'NONE', #11604 ) ;
#10599=EDGE_LOOP ( 'NONE', ( #9032, #545, #365, #12121 ) ) ;
#10605=EDGE_CURVE ( 'NONE', #5042, #69, #11663, .T. ) ;
#10647=ORIENTED_EDGE ( 'NONE', *, *, #10564, .F. ) ;
#10649=EDGE_CURVE ( 'NONE', #5163, #1219, #1927, .T. ) ;
#10686=EDGE_CURVE ( 'NONE', #8172, #5876, #11227, .T. ) ;
#10691=VECTOR ( 'NONE', #5057, 1000.000000000000000 ) ;
#10719=ORIENTED_EDGE ( 'NONE', *, *, #10735, .F. ) ;
#10735=EDGE_CURVE ( 'NONE', #2073, #10209, #4493, .T. ) ;
#10747=DIRECTION ( 'NONE',  ( 0.000000000000000000, 0.000000000000000000, 1.000000000000000000 ) ) ;
#10782=CARTESIAN_POINT ( 'NONE',  ( 1.387778780781445676E-14, -6.000000000000000000, 126.4213562373094959 ) ) ;
#10802=DIRECTION ( 'NONE',  ( 0.000000000000000000, 0.000000000000000000, 1.000000000000000000 ) ) ;
#10831=DIRECTION ( 'NONE',  ( 0.000000000000000000, 0.000000000000000000, 1.000000000000000000 ) ) ;
#10882=ORIENTED_EDGE ( 'NONE', *, *, #3822, .F. ) ;
#10904=DIRECTION ( 'NONE',  ( 0.000000000000000000, 0.000000000000000000, 1.000000000000000000 ) ) ;
#10933=CARTESIAN_POINT ( 'NONE',  ( -6.360897667028196044E-14, -6.000000000000000000, -141.4213562373094817 ) ) ;
#10946=DIRECTION ( 'NONE',  ( 0.000000000000000000, 1.000000000000000000, 0.000000000000000000 ) ) ;
#10986=FACE_OUTER_BOUND ( 'NONE', #7722, .T. ) ;
#11001=CARTESIAN_POINT ( 'NONE',  ( 1.387778780781445676E-14, 0.000000000000000000, 126.4213562373094959 ) ) ;
#11005=CARTESIAN_POINT ( 'NONE',  ( 0.000000000000000000, 0.000000000000000000, 0.000000000000000000 ) ) ;
#11017=CARTESIAN_POINT ( 'NONE',  ( -6.360897667028196044E-14, -6.000000000000000000, -141.4213562373094817 ) ) ;
#11027=AXIS2_PLACEMENT_3D ( 'NONE', #405, #8830, #10802 ) ;
#11029=CARTESIAN_POINT ( 'NONE',  ( 126.4213562373094959, -6.000000000000000000, -6.938893903907228378E-15 ) ) ;
#11042=EDGE_CURVE ( 'NONE', #6737, #368, #81, .T. ) ;
#11070=PLANE ( 'NONE',  #5101 ) ;
#11071=CARTESIAN_POINT ( 'NONE',  ( 1.387778780781445676E-14, -6.000000000000000000, 133.9213562373095101 ) ) ;
#11092=CARTESIAN_POINT ( 'NONE',  ( -126.4213562373094959, 0.000000000000000000, 2.255140518769849223E-14 ) ) ;
#11104=DIRECTION ( 'NONE',  ( 0.000000000000000000, 1.000000000000000000, 0.000000000000000000 ) ) ;
#11130=DIRECTION ( 'NONE',  ( 0.000000000000000000, 0.000000000000000000, 1.000000000000000000 ) ) ;
#11168=ORIENTED_EDGE ( 'NONE', *, *, #10605, .T. ) ;
#11227=LINE ( 'NONE', #3407, #8248 ) ;
#11237=CARTESIAN_POINT ( 'NONE',  ( -141.4213562373095101, -6.000000000000000000, 3.644282033693712520E-14 ) ) ;
#11247=ORIENTED_EDGE ( 'NONE', *, *, #10064, .T. ) ;
#11248=FACE_OUTER_BOUND ( 'NONE', #5494, .T. ) ;
#11259=DIRECTION ( 'NONE',  ( 0.7071067811865473507, 0.000000000000000000, -0.7071067811865477948 ) ) ;
#11276=ORIENTED_EDGE ( 'NONE', *, *, #6542, .F. ) ;
#11311=EDGE_CURVE ( 'NONE', #8172, #206, #1284, .T. ) ;
#11333=CIRCLE ( 'NONE', #4823, 7.500000000000007105 ) ;
#11381=AXIS2_PLACEMENT_3D ( 'NONE', #5018, #4161, #7876 ) ;
#11392=VECTOR ( 'NONE', #10239, 1000.000000000000000 ) ;
#11412=DIRECTION ( 'NONE',  ( 0.000000000000000000, 1.000000000000000000, 0.000000000000000000 ) ) ;
#11418=CARTESIAN_POINT ( 'NONE',  ( -126.4213562373094959, 0.000000000000000000, 7.500000000000035527 ) ) ;
#11435=EDGE_LOOP ( 'NONE', ( #1436, #951 ) ) ;
#11443=ORIENTED_EDGE ( 'NONE', *, *, #11311, .T. ) ;
#11477=PRODUCT_DEFINITION_CONTEXT ( 'detailed design', #7158, 'design' ) ;
#11521=AXIS2_PLACEMENT_3D ( 'NONE', #6592, #11104, #6338 ) ;
#11558=CYLINDRICAL_SURFACE ( 'NONE', #5108, 7.500000000000007105 ) ;
#11595=ORIENTED_EDGE ( 'NONE', *, *, #3136, .F. ) ;
#11604=CARTESIAN_POINT ( 'NONE',  ( 0.000000000000000000, -6.000000000000000000, -118.9213562373094817 ) ) ;
#11663=LINE ( 'NONE', #6957, #7649 ) ;
#11666=SHAPE_REPRESENTATION_RELATIONSHIP ( 'NONE' , 'NONE' ,  #2032, #8841 ) ;
#11685=CARTESIAN_POINT ( 'NONE',  ( 126.4213562373094959, -6.000000000000000000, -7.500000000000019540 ) ) ;
#11692=EDGE_CURVE ( 'NONE', #10573, #1414, #8304, .T. ) ;
#11723=EDGE_LOOP ( 'NONE', ( #10250, #10882 ) ) ;
#11782=VERTEX_POINT ( 'NONE', #3709 ) ;
#11805=DIRECTION ( 'NONE',  ( 0.000000000000000000, 0.000000000000000000, 1.000000000000000000 ) ) ;
#11814=CIRCLE ( 'NONE', #760, 7.500000000000012434 ) ;
#11833=CARTESIAN_POINT ( 'NONE',  ( -141.4213562373095101, -6.000000000000000000, 3.644282033693712520E-14 ) ) ;
#11844=ORIENTED_EDGE ( 'NONE', *, *, #11692, .F. ) ;
#11846=LINE ( 'NONE', #715, #8009 ) ;
#11867=DIRECTION ( 'NONE',  ( 0.000000000000000000, 1.000000000000000000, 0.000000000000000000 ) ) ;
#11929=VECTOR ( 'NONE', #11259, 999.9999999999998863 ) ;
#11946=CARTESIAN_POINT ( 'NONE',  ( 126.4213562373094959, -6.000000000000000000, -6.938893903907228378E-15 ) ) ;
#11957=AXIS2_PLACEMENT_3D ( 'NONE', #9048, #10904, #7955 ) ;
#11968=DIRECTION ( 'NONE',  ( 0.7071067811865479058, 0.000000000000000000, 0.7071067811865472397 ) ) ;
#11986=EDGE_CURVE ( 'NONE', #5042, #2268, #11846, .T. ) ;
#11994=CARTESIAN_POINT ( 'NONE',  ( 126.4213562373094959, 0.000000000000000000, -6.938893903907228378E-15 ) ) ;
#12001=VERTEX_POINT ( 'NONE', #6333 ) ;
#12003=ORIENTED_EDGE ( 'NONE', *, *, #238, .F. ) ;
#12008=CYLINDRICAL_SURFACE ( 'NONE', #4977, 7.500000000000012434 ) ;
#12009=ORIENTED_EDGE ( 'NONE', *, *, #4965, .F. ) ;
#12037=ORIENTED_EDGE ( 'NONE', *, *, #10064, .F. ) ;
#12111=DIRECTION ( 'NONE',  ( 0.000000000000000000, 1.000000000000000000, 0.000000000000000000 ) ) ;
#12120=AXIS2_PLACEMENT_3D ( 'NONE', #8823, #5540, #11968 ) ;
#12121=ORIENTED_EDGE ( 'NONE', *, *, #3803, .T. ) ;
#12124=CARTESIAN_POINT ( 'NONE',  ( 4.808665244885994618E-14, 0.000000000000000000, 141.4213562373094817 ) ) ;
#12129=ORIENTED_EDGE ( 'NONE', *, *, #3563, .T. ) ;
#12132=AXIS2_PLACEMENT_3D ( 'NONE', #2723, #617, #7236 ) ;
#12189=CARTESIAN_POINT ( 'NONE',  ( 126.4213562373094959, 0.000000000000000000, -6.938893903907228378E-15 ) ) ;
#12195=FACE_OUTER_BOUND ( 'NONE', #809, .T. ) ;
#12235=AXIS2_PLACEMENT_3D ( 'NONE', #11001, #11867, #10072 ) ;
ENDSEC;
END-ISO-10303-21;
